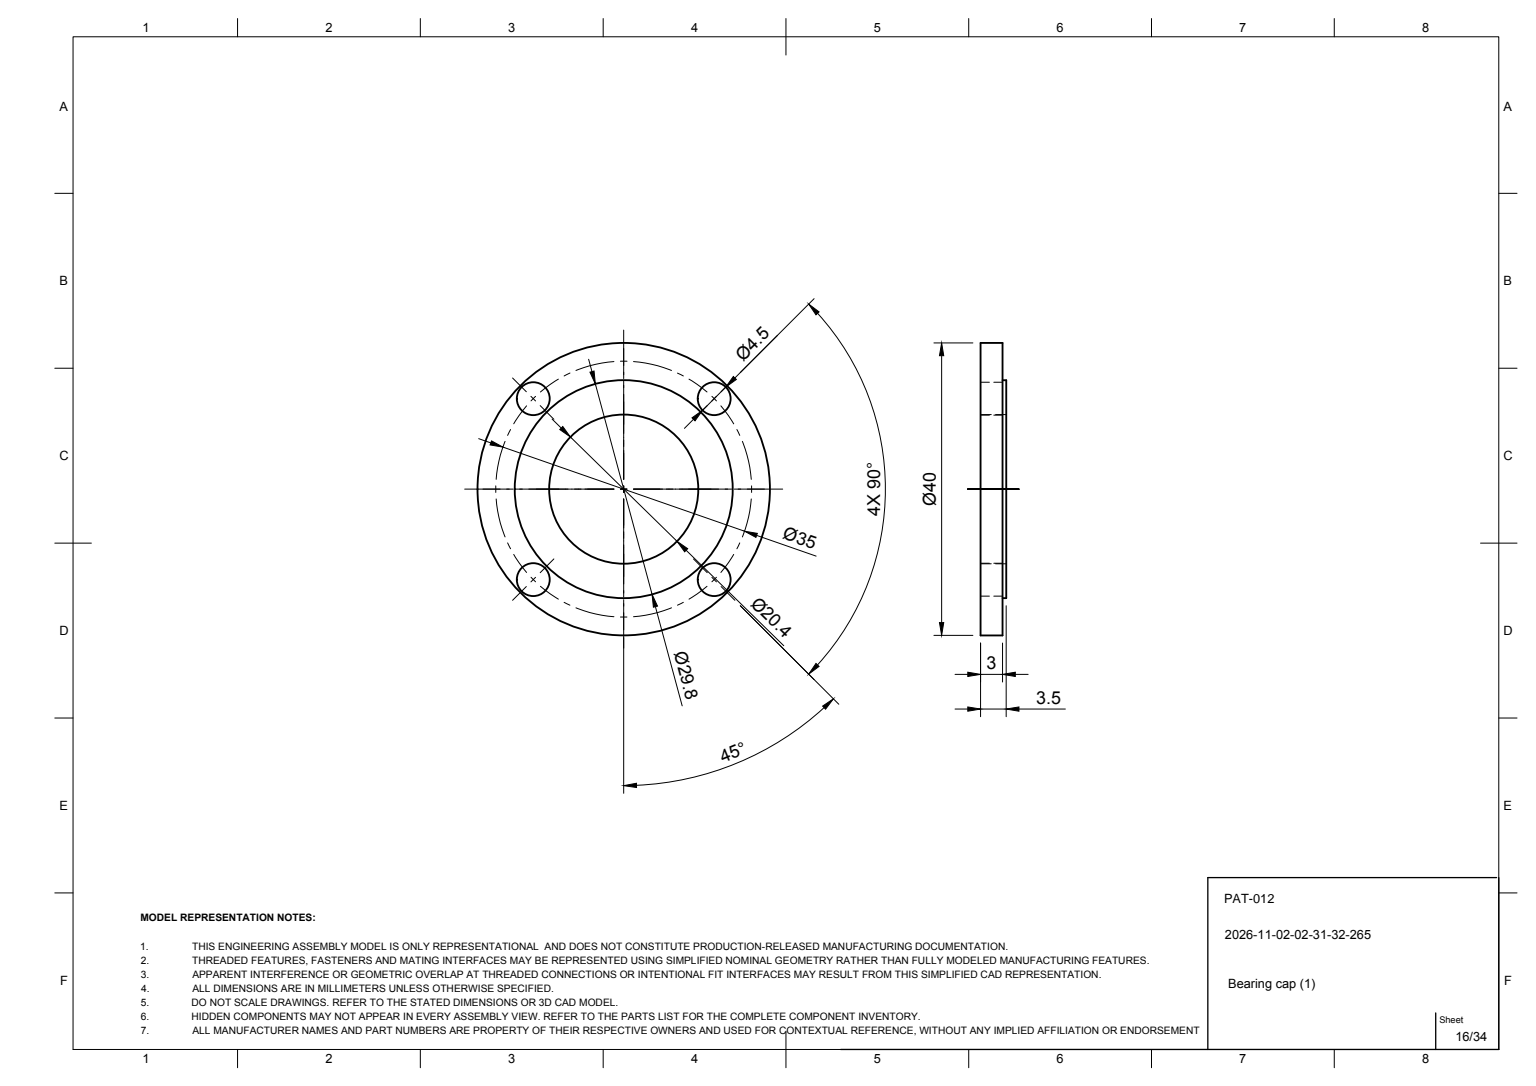
ISO-10303-21;
HEADER;
/* Generated by software containing ST-Developer
 * from STEP Tools, Inc. (www.steptools.com) 
 */

FILE_DESCRIPTION(
/* description */ ('Belt tensioner idler arm'),
/* implementation_level */ '2;1');

FILE_NAME(
/* name */ 'Bearing cap (1).step',
/* time_stamp */ '2026-10-28T03:22:15-07:00',
/* author */ (''),
/* organization */ (''),
/* preprocessor_version */ 'ST-DEVELOPER v20.2',
/* originating_system */ 'Autodesk Translation Framework v15.17.0.0',
/* authorisation */ '');

FILE_SCHEMA (('AUTOMOTIVE_DESIGN { 1 0 10303 214 3 1 1 }'));
ENDSEC;

DATA;
#10=MECHANICAL_DESIGN_GEOMETRIC_PRESENTATION_REPRESENTATION('',(#461),#12779);
#393=SHAPE_REPRESENTATION_RELATIONSHIP('SRR','None',#12940,#427);
#427=ADVANCED_BREP_SHAPE_REPRESENTATION('',(#501),#12757);
#461=STYLED_ITEM('',(#13184),#501);
#501=MANIFOLD_SOLID_BREP('Body1',#6197);
#593=FACE_BOUND('',#1421,.T.);
#594=FACE_BOUND('',#1425,.T.);
#595=FACE_BOUND('',#1426,.T.);
#596=FACE_BOUND('',#1427,.T.);
#597=FACE_BOUND('',#1428,.T.);
#598=FACE_BOUND('',#1429,.T.);
#599=FACE_BOUND('',#1431,.T.);
#600=FACE_BOUND('',#1432,.T.);
#601=FACE_BOUND('',#1433,.T.);
#602=FACE_BOUND('',#1434,.T.);
#603=FACE_BOUND('',#1435,.T.);
#747=PLANE('',#6891);
#748=PLANE('',#6898);
#749=PLANE('',#6899);
#982=FACE_OUTER_BOUND('',#1415,.T.);
#983=FACE_OUTER_BOUND('',#1416,.T.);
#984=FACE_OUTER_BOUND('',#1417,.T.);
#985=FACE_OUTER_BOUND('',#1418,.T.);
#986=FACE_OUTER_BOUND('',#1419,.T.);
#987=FACE_OUTER_BOUND('',#1420,.T.);
#988=FACE_OUTER_BOUND('',#1422,.T.);
#989=FACE_OUTER_BOUND('',#1423,.T.);
#990=FACE_OUTER_BOUND('',#1424,.T.);
#991=FACE_OUTER_BOUND('',#1430,.T.);
#1415=EDGE_LOOP('',(#4680,#4681,#4682,#4683));
#1416=EDGE_LOOP('',(#4684,#4685,#4686,#4687));
#1417=EDGE_LOOP('',(#4688,#4689,#4690,#4691));
#1418=EDGE_LOOP('',(#4692,#4693,#4694,#4695));
#1419=EDGE_LOOP('',(#4696,#4697,#4698,#4699));
#1420=EDGE_LOOP('',(#4700));
#1421=EDGE_LOOP('',(#4701));
#1422=EDGE_LOOP('',(#4702,#4703,#4704,#4705));
#1423=EDGE_LOOP('',(#4706,#4707,#4708,#4709));
#1424=EDGE_LOOP('',(#4710));
#1425=EDGE_LOOP('',(#4711));
#1426=EDGE_LOOP('',(#4712));
#1427=EDGE_LOOP('',(#4713));
#1428=EDGE_LOOP('',(#4714));
#1429=EDGE_LOOP('',(#4715));
#1430=EDGE_LOOP('',(#4716));
#1431=EDGE_LOOP('',(#4717));
#1432=EDGE_LOOP('',(#4718));
#1433=EDGE_LOOP('',(#4719));
#1434=EDGE_LOOP('',(#4720));
#1435=EDGE_LOOP('',(#4721));
#1868=LINE('',#10826,#2217);
#1869=LINE('',#10832,#2218);
#1870=LINE('',#10838,#2219);
#1871=LINE('',#10844,#2220);
#1872=LINE('',#10850,#2221);
#1873=LINE('',#10858,#2222);
#1874=LINE('',#10863,#2223);
#2217=VECTOR('',#8146,0.225);
#2218=VECTOR('',#8153,0.225);
#2219=VECTOR('',#8160,0.225);
#2220=VECTOR('',#8167,0.225);
#2221=VECTOR('',#8174,1.49);
#2222=VECTOR('',#8185,1.02);
#2223=VECTOR('',#8190,2.);
#2516=CIRCLE('',#6877,0.225);
#2517=CIRCLE('',#6878,0.225);
#2518=CIRCLE('',#6880,0.225);
#2519=CIRCLE('',#6881,0.225);
#2520=CIRCLE('',#6883,0.225);
#2521=CIRCLE('',#6884,0.225);
#2522=CIRCLE('',#6886,0.225);
#2523=CIRCLE('',#6887,0.225);
#2524=CIRCLE('',#6889,1.49);
#2525=CIRCLE('',#6890,1.49);
#2526=CIRCLE('',#6892,1.02);
#2527=CIRCLE('',#6894,1.02);
#2528=CIRCLE('',#6896,2.);
#2529=CIRCLE('',#6897,2.);
#2961=VERTEX_POINT('',#10823);
#2962=VERTEX_POINT('',#10825);
#2963=VERTEX_POINT('',#10829);
#2964=VERTEX_POINT('',#10831);
#2965=VERTEX_POINT('',#10835);
#2966=VERTEX_POINT('',#10837);
#2967=VERTEX_POINT('',#10841);
#2968=VERTEX_POINT('',#10843);
#2969=VERTEX_POINT('',#10847);
#2970=VERTEX_POINT('',#10849);
#2971=VERTEX_POINT('',#10853);
#2972=VERTEX_POINT('',#10856);
#2973=VERTEX_POINT('',#10860);
#2974=VERTEX_POINT('',#10862);
#3595=EDGE_CURVE('',#2961,#2961,#2516,.T.);
#3596=EDGE_CURVE('',#2961,#2962,#1868,.T.);
#3597=EDGE_CURVE('',#2962,#2962,#2517,.T.);
#3598=EDGE_CURVE('',#2963,#2963,#2518,.T.);
#3599=EDGE_CURVE('',#2963,#2964,#1869,.T.);
#3600=EDGE_CURVE('',#2964,#2964,#2519,.T.);
#3601=EDGE_CURVE('',#2965,#2965,#2520,.T.);
#3602=EDGE_CURVE('',#2965,#2966,#1870,.T.);
#3603=EDGE_CURVE('',#2966,#2966,#2521,.T.);
#3604=EDGE_CURVE('',#2967,#2967,#2522,.T.);
#3605=EDGE_CURVE('',#2967,#2968,#1871,.T.);
#3606=EDGE_CURVE('',#2968,#2968,#2523,.T.);
#3607=EDGE_CURVE('',#2969,#2969,#2524,.T.);
#3608=EDGE_CURVE('',#2969,#2970,#1872,.T.);
#3609=EDGE_CURVE('',#2970,#2970,#2525,.T.);
#3610=EDGE_CURVE('',#2971,#2971,#2526,.T.);
#3611=EDGE_CURVE('',#2972,#2972,#2527,.T.);
#3612=EDGE_CURVE('',#2972,#2971,#1873,.T.);
#3613=EDGE_CURVE('',#2973,#2973,#2528,.T.);
#3614=EDGE_CURVE('',#2973,#2974,#1874,.T.);
#3615=EDGE_CURVE('',#2974,#2974,#2529,.T.);
#4680=ORIENTED_EDGE('',*,*,#3595,.F.);
#4681=ORIENTED_EDGE('',*,*,#3596,.T.);
#4682=ORIENTED_EDGE('',*,*,#3597,.F.);
#4683=ORIENTED_EDGE('',*,*,#3596,.F.);
#4684=ORIENTED_EDGE('',*,*,#3598,.F.);
#4685=ORIENTED_EDGE('',*,*,#3599,.T.);
#4686=ORIENTED_EDGE('',*,*,#3600,.F.);
#4687=ORIENTED_EDGE('',*,*,#3599,.F.);
#4688=ORIENTED_EDGE('',*,*,#3601,.F.);
#4689=ORIENTED_EDGE('',*,*,#3602,.T.);
#4690=ORIENTED_EDGE('',*,*,#3603,.F.);
#4691=ORIENTED_EDGE('',*,*,#3602,.F.);
#4692=ORIENTED_EDGE('',*,*,#3604,.F.);
#4693=ORIENTED_EDGE('',*,*,#3605,.T.);
#4694=ORIENTED_EDGE('',*,*,#3606,.F.);
#4695=ORIENTED_EDGE('',*,*,#3605,.F.);
#4696=ORIENTED_EDGE('',*,*,#3607,.F.);
#4697=ORIENTED_EDGE('',*,*,#3608,.T.);
#4698=ORIENTED_EDGE('',*,*,#3609,.T.);
#4699=ORIENTED_EDGE('',*,*,#3608,.F.);
#4700=ORIENTED_EDGE('',*,*,#3609,.F.);
#4701=ORIENTED_EDGE('',*,*,#3610,.F.);
#4702=ORIENTED_EDGE('',*,*,#3611,.F.);
#4703=ORIENTED_EDGE('',*,*,#3612,.T.);
#4704=ORIENTED_EDGE('',*,*,#3610,.T.);
#4705=ORIENTED_EDGE('',*,*,#3612,.F.);
#4706=ORIENTED_EDGE('',*,*,#3613,.F.);
#4707=ORIENTED_EDGE('',*,*,#3614,.T.);
#4708=ORIENTED_EDGE('',*,*,#3615,.T.);
#4709=ORIENTED_EDGE('',*,*,#3614,.F.);
#4710=ORIENTED_EDGE('',*,*,#3613,.T.);
#4711=ORIENTED_EDGE('',*,*,#3611,.T.);
#4712=ORIENTED_EDGE('',*,*,#3606,.T.);
#4713=ORIENTED_EDGE('',*,*,#3603,.T.);
#4714=ORIENTED_EDGE('',*,*,#3600,.T.);
#4715=ORIENTED_EDGE('',*,*,#3597,.T.);
#4716=ORIENTED_EDGE('',*,*,#3615,.F.);
#4717=ORIENTED_EDGE('',*,*,#3607,.T.);
#4718=ORIENTED_EDGE('',*,*,#3604,.T.);
#4719=ORIENTED_EDGE('',*,*,#3601,.T.);
#4720=ORIENTED_EDGE('',*,*,#3598,.T.);
#4721=ORIENTED_EDGE('',*,*,#3595,.T.);
#5711=CYLINDRICAL_SURFACE('',#6876,0.225);
#5712=CYLINDRICAL_SURFACE('',#6879,0.225);
#5713=CYLINDRICAL_SURFACE('',#6882,0.225);
#5714=CYLINDRICAL_SURFACE('',#6885,0.225);
#5715=CYLINDRICAL_SURFACE('',#6888,1.49);
#5716=CYLINDRICAL_SURFACE('',#6893,1.02);
#5717=CYLINDRICAL_SURFACE('',#6895,2.);
#5959=ADVANCED_FACE('',(#982),#5711,.F.);
#5960=ADVANCED_FACE('',(#983),#5712,.F.);
#5961=ADVANCED_FACE('',(#984),#5713,.F.);
#5962=ADVANCED_FACE('',(#985),#5714,.F.);
#5963=ADVANCED_FACE('',(#986),#5715,.T.);
#5964=ADVANCED_FACE('',(#987,#593),#747,.F.);
#5965=ADVANCED_FACE('',(#988),#5716,.F.);
#5966=ADVANCED_FACE('',(#989),#5717,.T.);
#5967=ADVANCED_FACE('',(#990,#594,#595,#596,#597,#598),#748,.T.);
#5968=ADVANCED_FACE('',(#991,#599,#600,#601,#602,#603),#749,.F.);
#6197=CLOSED_SHELL('',(#5959,#5960,#5961,#5962,#5963,#5964,#5965,#5966,
#5967,#5968));
#6875=AXIS2_PLACEMENT_3D('',#10821,#8140,#8141);
#6876=AXIS2_PLACEMENT_3D('',#10822,#8142,#8143);
#6877=AXIS2_PLACEMENT_3D('',#10824,#8144,#8145);
#6878=AXIS2_PLACEMENT_3D('',#10827,#8147,#8148);
#6879=AXIS2_PLACEMENT_3D('',#10828,#8149,#8150);
#6880=AXIS2_PLACEMENT_3D('',#10830,#8151,#8152);
#6881=AXIS2_PLACEMENT_3D('',#10833,#8154,#8155);
#6882=AXIS2_PLACEMENT_3D('',#10834,#8156,#8157);
#6883=AXIS2_PLACEMENT_3D('',#10836,#8158,#8159);
#6884=AXIS2_PLACEMENT_3D('',#10839,#8161,#8162);
#6885=AXIS2_PLACEMENT_3D('',#10840,#8163,#8164);
#6886=AXIS2_PLACEMENT_3D('',#10842,#8165,#8166);
#6887=AXIS2_PLACEMENT_3D('',#10845,#8168,#8169);
#6888=AXIS2_PLACEMENT_3D('',#10846,#8170,#8171);
#6889=AXIS2_PLACEMENT_3D('',#10848,#8172,#8173);
#6890=AXIS2_PLACEMENT_3D('',#10851,#8175,#8176);
#6891=AXIS2_PLACEMENT_3D('',#10852,#8177,#8178);
#6892=AXIS2_PLACEMENT_3D('',#10854,#8179,#8180);
#6893=AXIS2_PLACEMENT_3D('',#10855,#8181,#8182);
#6894=AXIS2_PLACEMENT_3D('',#10857,#8183,#8184);
#6895=AXIS2_PLACEMENT_3D('',#10859,#8186,#8187);
#6896=AXIS2_PLACEMENT_3D('',#10861,#8188,#8189);
#6897=AXIS2_PLACEMENT_3D('',#10864,#8191,#8192);
#6898=AXIS2_PLACEMENT_3D('',#10865,#8193,#8194);
#6899=AXIS2_PLACEMENT_3D('',#10866,#8195,#8196);
#8140=DIRECTION('axis',(0.,0.,1.));
#8141=DIRECTION('refdir',(1.,0.,0.));
#8142=DIRECTION('center_axis',(0.,0.,1.));
#8143=DIRECTION('ref_axis',(1.,0.,0.));
#8144=DIRECTION('center_axis',(0.,0.,1.));
#8145=DIRECTION('ref_axis',(1.,0.,0.));
#8146=DIRECTION('',(0.,0.,1.));
#8147=DIRECTION('center_axis',(0.,0.,-1.));
#8148=DIRECTION('ref_axis',(1.,0.,0.));
#8149=DIRECTION('center_axis',(0.,0.,1.));
#8150=DIRECTION('ref_axis',(1.,0.,0.));
#8151=DIRECTION('center_axis',(0.,0.,1.));
#8152=DIRECTION('ref_axis',(1.,0.,0.));
#8153=DIRECTION('',(0.,0.,1.));
#8154=DIRECTION('center_axis',(0.,0.,-1.));
#8155=DIRECTION('ref_axis',(1.,0.,0.));
#8156=DIRECTION('center_axis',(0.,0.,1.));
#8157=DIRECTION('ref_axis',(1.,0.,0.));
#8158=DIRECTION('center_axis',(0.,0.,1.));
#8159=DIRECTION('ref_axis',(1.,0.,0.));
#8160=DIRECTION('',(0.,0.,1.));
#8161=DIRECTION('center_axis',(0.,0.,-1.));
#8162=DIRECTION('ref_axis',(1.,0.,0.));
#8163=DIRECTION('center_axis',(0.,0.,1.));
#8164=DIRECTION('ref_axis',(1.,0.,0.));
#8165=DIRECTION('center_axis',(0.,0.,1.));
#8166=DIRECTION('ref_axis',(1.,0.,0.));
#8167=DIRECTION('',(0.,0.,1.));
#8168=DIRECTION('center_axis',(0.,0.,-1.));
#8169=DIRECTION('ref_axis',(1.,0.,0.));
#8170=DIRECTION('center_axis',(0.,0.,1.));
#8171=DIRECTION('ref_axis',(1.,0.,0.));
#8172=DIRECTION('center_axis',(0.,0.,1.));
#8173=DIRECTION('ref_axis',(1.,0.,0.));
#8174=DIRECTION('',(0.,0.,-1.));
#8175=DIRECTION('center_axis',(0.,0.,1.));
#8176=DIRECTION('ref_axis',(1.,0.,0.));
#8177=DIRECTION('center_axis',(0.,0.,1.));
#8178=DIRECTION('ref_axis',(1.,0.,0.));
#8179=DIRECTION('center_axis',(0.,0.,-1.));
#8180=DIRECTION('ref_axis',(1.,0.,0.));
#8181=DIRECTION('center_axis',(0.,0.,1.));
#8182=DIRECTION('ref_axis',(1.,0.,0.));
#8183=DIRECTION('center_axis',(0.,0.,-1.));
#8184=DIRECTION('ref_axis',(1.,0.,0.));
#8185=DIRECTION('',(0.,0.,-1.));
#8186=DIRECTION('center_axis',(0.,0.,1.));
#8187=DIRECTION('ref_axis',(1.,0.,0.));
#8188=DIRECTION('center_axis',(0.,0.,1.));
#8189=DIRECTION('ref_axis',(1.,0.,0.));
#8190=DIRECTION('',(0.,0.,-1.));
#8191=DIRECTION('center_axis',(0.,0.,1.));
#8192=DIRECTION('ref_axis',(1.,0.,0.));
#8193=DIRECTION('center_axis',(0.,0.,1.));
#8194=DIRECTION('ref_axis',(1.,0.,0.));
#8195=DIRECTION('center_axis',(0.,0.,1.));
#8196=DIRECTION('ref_axis',(1.,0.,0.));
#10821=CARTESIAN_POINT('',(0.,0.,0.));
#10822=CARTESIAN_POINT('Origin',(-1.23743686707646,-1.23743686707646,5.9));
#10823=CARTESIAN_POINT('',(-1.46243686707646,-1.23743686707646,6.));
#10824=CARTESIAN_POINT('Origin',(-1.23743686707646,-1.23743686707646,6.));
#10825=CARTESIAN_POINT('',(-1.46243686707646,-1.23743686707646,6.3));
#10826=CARTESIAN_POINT('',(-1.46243686707646,-1.23743686707646,5.9));
#10827=CARTESIAN_POINT('Origin',(-1.23743686707646,-1.23743686707646,6.3));
#10828=CARTESIAN_POINT('Origin',(-1.23743686707646,1.23743686707646,5.9));
#10829=CARTESIAN_POINT('',(-1.46243686707646,1.23743686707646,6.));
#10830=CARTESIAN_POINT('Origin',(-1.23743686707646,1.23743686707646,6.));
#10831=CARTESIAN_POINT('',(-1.46243686707646,1.23743686707646,6.3));
#10832=CARTESIAN_POINT('',(-1.46243686707646,1.23743686707646,5.9));
#10833=CARTESIAN_POINT('Origin',(-1.23743686707646,1.23743686707646,6.3));
#10834=CARTESIAN_POINT('Origin',(1.23743686707646,1.23743686707646,5.9));
#10835=CARTESIAN_POINT('',(1.01243686707646,1.23743686707646,6.));
#10836=CARTESIAN_POINT('Origin',(1.23743686707646,1.23743686707646,6.));
#10837=CARTESIAN_POINT('',(1.01243686707646,1.23743686707646,6.3));
#10838=CARTESIAN_POINT('',(1.01243686707646,1.23743686707646,5.9));
#10839=CARTESIAN_POINT('Origin',(1.23743686707646,1.23743686707646,6.3));
#10840=CARTESIAN_POINT('Origin',(1.23743686707646,-1.23743686707646,5.9));
#10841=CARTESIAN_POINT('',(1.01243686707646,-1.23743686707646,6.));
#10842=CARTESIAN_POINT('Origin',(1.23743686707646,-1.23743686707646,6.));
#10843=CARTESIAN_POINT('',(1.01243686707646,-1.23743686707646,6.3));
#10844=CARTESIAN_POINT('',(1.01243686707646,-1.23743686707646,5.9));
#10845=CARTESIAN_POINT('Origin',(1.23743686707646,-1.23743686707646,6.3));
#10846=CARTESIAN_POINT('Origin',(0.,0.,5.95));
#10847=CARTESIAN_POINT('',(-1.49,-1.82472373072956E-16,6.));
#10848=CARTESIAN_POINT('Origin',(0.,0.,6.));
#10849=CARTESIAN_POINT('',(-1.49,-1.82472373072956E-16,5.95));
#10850=CARTESIAN_POINT('',(-1.49,-1.82472373072956E-16,5.95));
#10851=CARTESIAN_POINT('Origin',(0.,0.,5.95));
#10852=CARTESIAN_POINT('Origin',(0.,0.,5.95));
#10853=CARTESIAN_POINT('',(-1.02,-1.2491397351303E-16,5.95));
#10854=CARTESIAN_POINT('Origin',(0.,0.,5.95));
#10855=CARTESIAN_POINT('Origin',(0.,0.,6.));
#10856=CARTESIAN_POINT('',(-1.02,-1.2491397351303E-16,6.3));
#10857=CARTESIAN_POINT('Origin',(0.,0.,6.3));
#10858=CARTESIAN_POINT('',(-1.02,-1.2491397351303E-16,6.));
#10859=CARTESIAN_POINT('Origin',(0.,0.,6.));
#10860=CARTESIAN_POINT('',(-2.,-2.44929359829471E-16,6.3));
#10861=CARTESIAN_POINT('Origin',(0.,0.,6.3));
#10862=CARTESIAN_POINT('',(-2.,-2.44929359829471E-16,6.));
#10863=CARTESIAN_POINT('',(-2.,-2.44929359829471E-16,6.));
#10864=CARTESIAN_POINT('Origin',(0.,0.,6.));
#10865=CARTESIAN_POINT('Origin',(0.,0.,6.3));
#10866=CARTESIAN_POINT('Origin',(0.,0.,6.));
#12717=UNCERTAINTY_MEASURE_WITH_UNIT(LENGTH_MEASURE(0.001),#12780,
'DISTANCE_ACCURACY_VALUE',
'Maximum model space distance between geometric entities at asserted c
onnectivities');
#12739=UNCERTAINTY_MEASURE_WITH_UNIT(LENGTH_MEASURE(0.001),#12780,
'DISTANCE_ACCURACY_VALUE',
'Maximum model space distance between geometric entities at asserted c
onnectivities');
#12757=(
GEOMETRIC_REPRESENTATION_CONTEXT(3)
GLOBAL_UNCERTAINTY_ASSIGNED_CONTEXT((#12717))
GLOBAL_UNIT_ASSIGNED_CONTEXT((#12780,#12782,#12783))
REPRESENTATION_CONTEXT('','3D')
);
#12779=(
GEOMETRIC_REPRESENTATION_CONTEXT(3)
GLOBAL_UNCERTAINTY_ASSIGNED_CONTEXT((#12739))
GLOBAL_UNIT_ASSIGNED_CONTEXT((#12780,#12782,#12783))
REPRESENTATION_CONTEXT('','3D')
);
#12780=(
LENGTH_UNIT()
NAMED_UNIT(*)
SI_UNIT(.CENTI.,.METRE.)
);
#12782=(
NAMED_UNIT(*)
PLANE_ANGLE_UNIT()
SI_UNIT($,.RADIAN.)
);
#12783=(
NAMED_UNIT(*)
SI_UNIT($,.STERADIAN.)
SOLID_ANGLE_UNIT()
);
#12801=SHAPE_DEFINITION_REPRESENTATION(#12840,#12940);
#12840=PRODUCT_DEFINITION_SHAPE('',$,#12980);
#12940=SHAPE_REPRESENTATION('',(#6875),#12757);
#12962=PRODUCT_DEFINITION_CONTEXT('part definition',#13081,'design');
#12980=PRODUCT_DEFINITION('Bearing cap (1)','Bearing cap (1)',#13019,#12962);
#13019=PRODUCT_DEFINITION_FORMATION('',$,#13100);
#13081=APPLICATION_CONTEXT(
'Core Data for Automotive Mechanical Design Process');
#13082=PRODUCT_CONTEXT('part definition',#13081,'mechanical');
#13100=PRODUCT('Bearing cap (1)','Bearing cap (1)','Bearing cap (1)',(#13082));
#13178=COLOUR_RGB('Grey',0.48,0.52,0.57);
#13179=FILL_AREA_STYLE_COLOUR('',#13178);
#13180=FILL_AREA_STYLE('',(#13179));
#13181=SURFACE_STYLE_FILL_AREA(#13180);
#13182=SURFACE_SIDE_STYLE('',(#13181));
#13183=SURFACE_STYLE_USAGE(.BOTH.,#13182);
#13184=PRESENTATION_STYLE_ASSIGNMENT((#13183));
ENDSEC;
END-ISO-10303-21;
